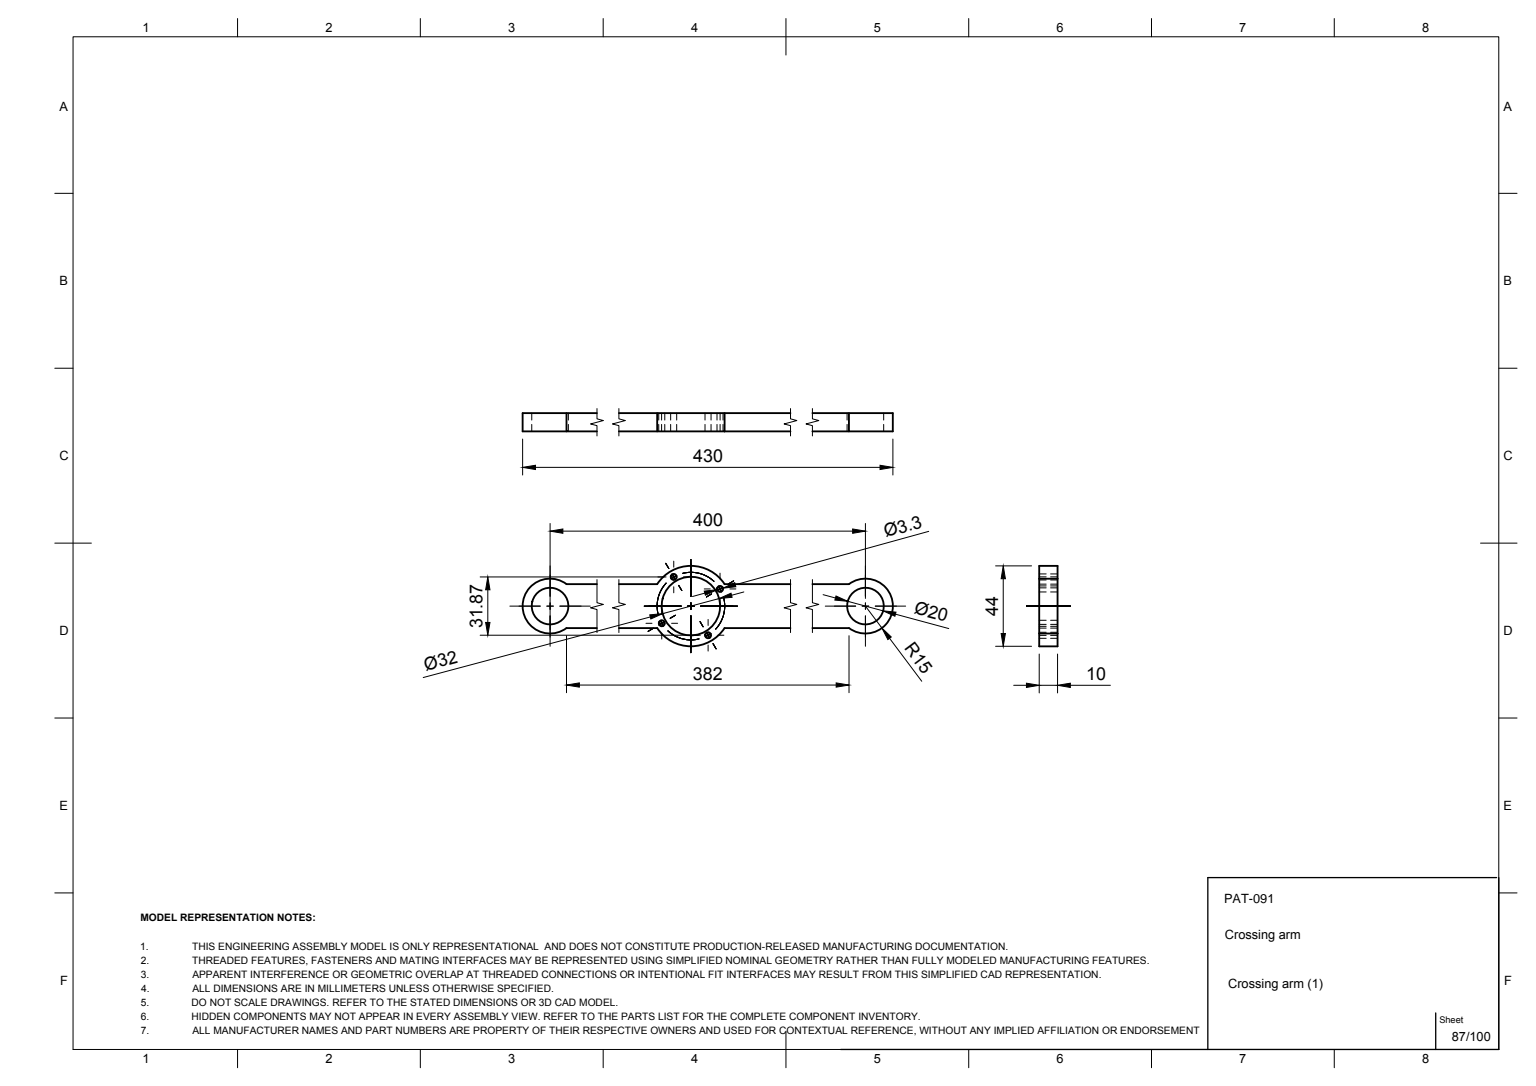
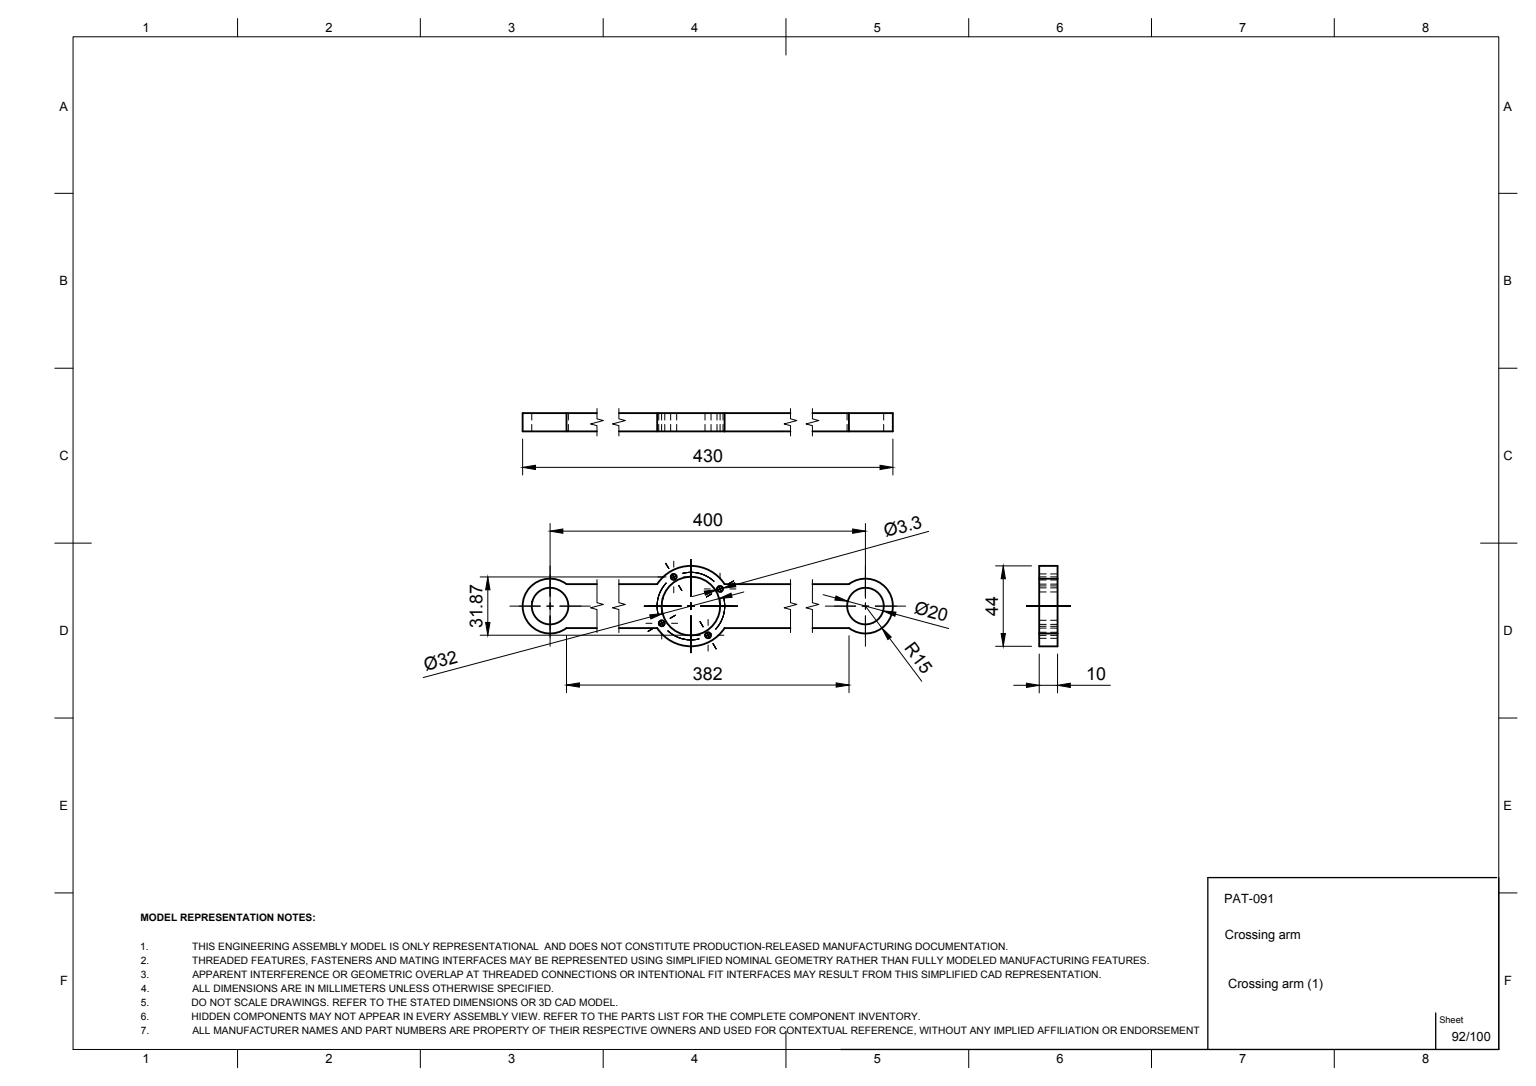
ISO-10303-21;
HEADER;
/* Generated by software containing ST-Developer
 * from STEP Tools, Inc. (www.steptools.com) 
 */

FILE_DESCRIPTION(
/* description */ ('PAT-091'),
/* implementation_level */ '2;1');

FILE_NAME(
/* name */ 'Crossing arm.step',
/* time_stamp */ '2026-10-27T15:34:44-07:00',
/* author */ (''),
/* organization */ (''),
/* preprocessor_version */ 'ST-DEVELOPER v20.2',
/* originating_system */ 'Autodesk Translation Framework v15.17.0.0',
/* authorisation */ '');

FILE_SCHEMA (('AUTOMOTIVE_DESIGN { 1 0 10303 214 3 1 1 }'));
ENDSEC;

DATA;
#10=MECHANICAL_DESIGN_GEOMETRIC_PRESENTATION_REPRESENTATION('',(#1044),#25100);
#824=SHAPE_REPRESENTATION_RELATIONSHIP('SRR','None',#25591,#934);
#934=ADVANCED_BREP_SHAPE_REPRESENTATION('',(#1165),#25061);
#1044=STYLED_ITEM('',(#26177),#1165);
#1165=MANIFOLD_SOLID_BREP('Body1',#13324);
#1525=FACE_BOUND('',#3750,.T.);
#1526=FACE_BOUND('',#3751,.T.);
#1527=FACE_BOUND('',#3752,.T.);
#1528=FACE_BOUND('',#3753,.T.);
#1529=FACE_BOUND('',#3754,.T.);
#1530=FACE_BOUND('',#3755,.T.);
#1531=FACE_BOUND('',#3756,.T.);
#1532=FACE_BOUND('',#3765,.T.);
#1533=FACE_BOUND('',#3766,.T.);
#1534=FACE_BOUND('',#3767,.T.);
#1535=FACE_BOUND('',#3768,.T.);
#1536=FACE_BOUND('',#3769,.T.);
#1537=FACE_BOUND('',#3770,.T.);
#1538=FACE_BOUND('',#3771,.T.);
#1948=PLANE('',#15794);
#1949=PLANE('',#15795);
#1950=PLANE('',#15800);
#1951=PLANE('',#15805);
#1952=PLANE('',#15810);
#1953=PLANE('',#15811);
#2613=FACE_OUTER_BOUND('',#3741,.T.);
#2614=FACE_OUTER_BOUND('',#3742,.T.);
#2615=FACE_OUTER_BOUND('',#3743,.T.);
#2616=FACE_OUTER_BOUND('',#3744,.T.);
#2617=FACE_OUTER_BOUND('',#3745,.T.);
#2618=FACE_OUTER_BOUND('',#3746,.T.);
#2619=FACE_OUTER_BOUND('',#3747,.T.);
#2620=FACE_OUTER_BOUND('',#3748,.T.);
#2621=FACE_OUTER_BOUND('',#3749,.T.);
#2622=FACE_OUTER_BOUND('',#3757,.T.);
#2623=FACE_OUTER_BOUND('',#3758,.T.);
#2624=FACE_OUTER_BOUND('',#3759,.T.);
#2625=FACE_OUTER_BOUND('',#3760,.T.);
#2626=FACE_OUTER_BOUND('',#3761,.T.);
#2627=FACE_OUTER_BOUND('',#3762,.T.);
#2628=FACE_OUTER_BOUND('',#3763,.T.);
#2629=FACE_OUTER_BOUND('',#3764,.T.);
#3741=EDGE_LOOP('',(#11144,#11145,#11146,#11147));
#3742=EDGE_LOOP('',(#11148,#11149,#11150,#11151));
#3743=EDGE_LOOP('',(#11152,#11153,#11154,#11155));
#3744=EDGE_LOOP('',(#11156,#11157,#11158,#11159));
#3745=EDGE_LOOP('',(#11160,#11161,#11162,#11163));
#3746=EDGE_LOOP('',(#11164,#11165,#11166,#11167));
#3747=EDGE_LOOP('',(#11168,#11169,#11170,#11171));
#3748=EDGE_LOOP('',(#11172,#11173,#11174,#11175));
#3749=EDGE_LOOP('',(#11176,#11177,#11178,#11179,#11180,#11181,#11182,#11183));
#3750=EDGE_LOOP('',(#11184));
#3751=EDGE_LOOP('',(#11185));
#3752=EDGE_LOOP('',(#11186));
#3753=EDGE_LOOP('',(#11187));
#3754=EDGE_LOOP('',(#11188));
#3755=EDGE_LOOP('',(#11189));
#3756=EDGE_LOOP('',(#11190));
#3757=EDGE_LOOP('',(#11191,#11192,#11193,#11194));
#3758=EDGE_LOOP('',(#11195,#11196,#11197,#11198));
#3759=EDGE_LOOP('',(#11199,#11200,#11201,#11202));
#3760=EDGE_LOOP('',(#11203,#11204,#11205,#11206));
#3761=EDGE_LOOP('',(#11207,#11208,#11209,#11210));
#3762=EDGE_LOOP('',(#11211,#11212,#11213,#11214));
#3763=EDGE_LOOP('',(#11215,#11216,#11217,#11218));
#3764=EDGE_LOOP('',(#11219,#11220,#11221,#11222,#11223,#11224,#11225,#11226));
#3765=EDGE_LOOP('',(#11227));
#3766=EDGE_LOOP('',(#11228));
#3767=EDGE_LOOP('',(#11229));
#3768=EDGE_LOOP('',(#11230));
#3769=EDGE_LOOP('',(#11231));
#3770=EDGE_LOOP('',(#11232));
#3771=EDGE_LOOP('',(#11233));
#4724=LINE('',#23542,#5464);
#4725=LINE('',#23548,#5465);
#4726=LINE('',#23554,#5466);
#4727=LINE('',#23560,#5467);
#4728=LINE('',#23566,#5468);
#4729=LINE('',#23571,#5469);
#4730=LINE('',#23575,#5470);
#4731=LINE('',#23580,#5471);
#4732=LINE('',#23584,#5472);
#4733=LINE('',#23588,#5473);
#4734=LINE('',#23590,#5474);
#4735=LINE('',#23591,#5475);
#4736=LINE('',#23595,#5476);
#4737=LINE('',#23597,#5477);
#4738=LINE('',#23600,#5478);
#4739=LINE('',#23607,#5479);
#4740=LINE('',#23608,#5480);
#4741=LINE('',#23612,#5481);
#4742=LINE('',#23615,#5482);
#4743=LINE('',#23618,#5483);
#4744=LINE('',#23620,#5484);
#4745=LINE('',#23624,#5485);
#4746=LINE('',#23628,#5486);
#5464=VECTOR('',#19448,0.164999999999999);
#5465=VECTOR('',#19455,0.164999999999999);
#5466=VECTOR('',#19462,0.164999999999999);
#5467=VECTOR('',#19469,0.164999999999999);
#5468=VECTOR('',#19476,1.6);
#5469=VECTOR('',#19481,1.);
#5470=VECTOR('',#19484,1.);
#5471=VECTOR('',#19489,1.);
#5472=VECTOR('',#19492,1.);
#5473=VECTOR('',#19497,1.);
#5474=VECTOR('',#19498,1.);
#5475=VECTOR('',#19499,1.);
#5476=VECTOR('',#19504,1.);
#5477=VECTOR('',#19505,1.);
#5478=VECTOR('',#19508,1.);
#5479=VECTOR('',#19515,1.);
#5480=VECTOR('',#19516,1.);
#5481=VECTOR('',#19521,1.);
#5482=VECTOR('',#19524,1.);
#5483=VECTOR('',#19527,1.);
#5484=VECTOR('',#19530,1.);
#5485=VECTOR('',#19535,1.);
#5486=VECTOR('',#19542,1.);
#6086=CIRCLE('',#15774,0.164999999999999);
#6087=CIRCLE('',#15775,0.164999999999999);
#6088=CIRCLE('',#15777,0.164999999999999);
#6089=CIRCLE('',#15778,0.164999999999999);
#6090=CIRCLE('',#15780,0.164999999999999);
#6091=CIRCLE('',#15781,0.164999999999999);
#6092=CIRCLE('',#15783,0.164999999999999);
#6093=CIRCLE('',#15784,0.164999999999999);
#6094=CIRCLE('',#15786,1.6);
#6095=CIRCLE('',#15787,1.6);
#6096=CIRCLE('',#15789,2.2);
#6097=CIRCLE('',#15790,2.2);
#6098=CIRCLE('',#15792,2.2);
#6099=CIRCLE('',#15793,2.2);
#6100=CIRCLE('',#15796,1.5);
#6101=CIRCLE('',#15797,1.5);
#6102=CIRCLE('',#15798,1.);
#6103=CIRCLE('',#15799,1.);
#6104=CIRCLE('',#15802,1.);
#6105=CIRCLE('',#15804,1.5);
#6106=CIRCLE('',#15807,1.);
#6107=CIRCLE('',#15809,1.5);
#7103=VERTEX_POINT('',#23539);
#7104=VERTEX_POINT('',#23541);
#7105=VERTEX_POINT('',#23545);
#7106=VERTEX_POINT('',#23547);
#7107=VERTEX_POINT('',#23551);
#7108=VERTEX_POINT('',#23553);
#7109=VERTEX_POINT('',#23557);
#7110=VERTEX_POINT('',#23559);
#7111=VERTEX_POINT('',#23563);
#7112=VERTEX_POINT('',#23565);
#7113=VERTEX_POINT('',#23569);
#7114=VERTEX_POINT('',#23570);
#7115=VERTEX_POINT('',#23572);
#7116=VERTEX_POINT('',#23574);
#7117=VERTEX_POINT('',#23578);
#7118=VERTEX_POINT('',#23579);
#7119=VERTEX_POINT('',#23581);
#7120=VERTEX_POINT('',#23583);
#7121=VERTEX_POINT('',#23587);
#7122=VERTEX_POINT('',#23589);
#7123=VERTEX_POINT('',#23593);
#7124=VERTEX_POINT('',#23596);
#7125=VERTEX_POINT('',#23598);
#7126=VERTEX_POINT('',#23601);
#7127=VERTEX_POINT('',#23603);
#7128=VERTEX_POINT('',#23606);
#7129=VERTEX_POINT('',#23610);
#7130=VERTEX_POINT('',#23614);
#7131=VERTEX_POINT('',#23616);
#7132=VERTEX_POINT('',#23622);
#8507=EDGE_CURVE('',#7103,#7103,#6086,.T.);
#8508=EDGE_CURVE('',#7103,#7104,#4724,.T.);
#8509=EDGE_CURVE('',#7104,#7104,#6087,.T.);
#8510=EDGE_CURVE('',#7105,#7105,#6088,.T.);
#8511=EDGE_CURVE('',#7105,#7106,#4725,.T.);
#8512=EDGE_CURVE('',#7106,#7106,#6089,.T.);
#8513=EDGE_CURVE('',#7107,#7107,#6090,.T.);
#8514=EDGE_CURVE('',#7107,#7108,#4726,.T.);
#8515=EDGE_CURVE('',#7108,#7108,#6091,.T.);
#8516=EDGE_CURVE('',#7109,#7109,#6092,.T.);
#8517=EDGE_CURVE('',#7109,#7110,#4727,.T.);
#8518=EDGE_CURVE('',#7110,#7110,#6093,.T.);
#8519=EDGE_CURVE('',#7111,#7111,#6094,.T.);
#8520=EDGE_CURVE('',#7111,#7112,#4728,.T.);
#8521=EDGE_CURVE('',#7112,#7112,#6095,.T.);
#8522=EDGE_CURVE('',#7113,#7114,#4729,.T.);
#8523=EDGE_CURVE('',#7115,#7113,#6096,.T.);
#8524=EDGE_CURVE('',#7116,#7115,#4730,.T.);
#8525=EDGE_CURVE('',#7116,#7114,#6097,.T.);
#8526=EDGE_CURVE('',#7117,#7118,#4731,.T.);
#8527=EDGE_CURVE('',#7117,#7119,#6098,.T.);
#8528=EDGE_CURVE('',#7120,#7119,#4732,.T.);
#8529=EDGE_CURVE('',#7118,#7120,#6099,.T.);
#8530=EDGE_CURVE('',#7119,#7121,#4733,.T.);
#8531=EDGE_CURVE('',#7121,#7122,#4734,.T.);
#8532=EDGE_CURVE('',#7120,#7122,#4735,.T.);
#8533=EDGE_CURVE('',#7122,#7123,#6100,.T.);
#8534=EDGE_CURVE('',#7123,#7115,#4736,.T.);
#8535=EDGE_CURVE('',#7113,#7124,#4737,.T.);
#8536=EDGE_CURVE('',#7124,#7125,#6101,.T.);
#8537=EDGE_CURVE('',#7125,#7118,#4738,.T.);
#8538=EDGE_CURVE('',#7126,#7126,#6102,.T.);
#8539=EDGE_CURVE('',#7127,#7127,#6103,.T.);
#8540=EDGE_CURVE('',#7123,#7128,#4739,.T.);
#8541=EDGE_CURVE('',#7128,#7116,#4740,.T.);
#8542=EDGE_CURVE('',#7129,#7129,#6104,.T.);
#8543=EDGE_CURVE('',#7129,#7126,#4741,.T.);
#8544=EDGE_CURVE('',#7130,#7124,#4742,.T.);
#8545=EDGE_CURVE('',#7130,#7131,#6105,.T.);
#8546=EDGE_CURVE('',#7125,#7131,#4743,.T.);
#8547=EDGE_CURVE('',#7114,#7130,#4744,.T.);
#8548=EDGE_CURVE('',#7132,#7132,#6106,.T.);
#8549=EDGE_CURVE('',#7132,#7127,#4745,.T.);
#8550=EDGE_CURVE('',#7121,#7128,#6107,.T.);
#8551=EDGE_CURVE('',#7131,#7117,#4746,.T.);
#11144=ORIENTED_EDGE('',*,*,#8507,.F.);
#11145=ORIENTED_EDGE('',*,*,#8508,.T.);
#11146=ORIENTED_EDGE('',*,*,#8509,.F.);
#11147=ORIENTED_EDGE('',*,*,#8508,.F.);
#11148=ORIENTED_EDGE('',*,*,#8510,.F.);
#11149=ORIENTED_EDGE('',*,*,#8511,.T.);
#11150=ORIENTED_EDGE('',*,*,#8512,.F.);
#11151=ORIENTED_EDGE('',*,*,#8511,.F.);
#11152=ORIENTED_EDGE('',*,*,#8513,.F.);
#11153=ORIENTED_EDGE('',*,*,#8514,.T.);
#11154=ORIENTED_EDGE('',*,*,#8515,.F.);
#11155=ORIENTED_EDGE('',*,*,#8514,.F.);
#11156=ORIENTED_EDGE('',*,*,#8516,.F.);
#11157=ORIENTED_EDGE('',*,*,#8517,.T.);
#11158=ORIENTED_EDGE('',*,*,#8518,.F.);
#11159=ORIENTED_EDGE('',*,*,#8517,.F.);
#11160=ORIENTED_EDGE('',*,*,#8519,.F.);
#11161=ORIENTED_EDGE('',*,*,#8520,.T.);
#11162=ORIENTED_EDGE('',*,*,#8521,.F.);
#11163=ORIENTED_EDGE('',*,*,#8520,.F.);
#11164=ORIENTED_EDGE('',*,*,#8522,.F.);
#11165=ORIENTED_EDGE('',*,*,#8523,.F.);
#11166=ORIENTED_EDGE('',*,*,#8524,.F.);
#11167=ORIENTED_EDGE('',*,*,#8525,.T.);
#11168=ORIENTED_EDGE('',*,*,#8526,.F.);
#11169=ORIENTED_EDGE('',*,*,#8527,.T.);
#11170=ORIENTED_EDGE('',*,*,#8528,.F.);
#11171=ORIENTED_EDGE('',*,*,#8529,.F.);
#11172=ORIENTED_EDGE('',*,*,#8528,.T.);
#11173=ORIENTED_EDGE('',*,*,#8530,.T.);
#11174=ORIENTED_EDGE('',*,*,#8531,.T.);
#11175=ORIENTED_EDGE('',*,*,#8532,.F.);
#11176=ORIENTED_EDGE('',*,*,#8532,.T.);
#11177=ORIENTED_EDGE('',*,*,#8533,.T.);
#11178=ORIENTED_EDGE('',*,*,#8534,.T.);
#11179=ORIENTED_EDGE('',*,*,#8523,.T.);
#11180=ORIENTED_EDGE('',*,*,#8535,.T.);
#11181=ORIENTED_EDGE('',*,*,#8536,.T.);
#11182=ORIENTED_EDGE('',*,*,#8537,.T.);
#11183=ORIENTED_EDGE('',*,*,#8529,.T.);
#11184=ORIENTED_EDGE('',*,*,#8538,.T.);
#11185=ORIENTED_EDGE('',*,*,#8539,.T.);
#11186=ORIENTED_EDGE('',*,*,#8521,.T.);
#11187=ORIENTED_EDGE('',*,*,#8518,.T.);
#11188=ORIENTED_EDGE('',*,*,#8515,.T.);
#11189=ORIENTED_EDGE('',*,*,#8512,.T.);
#11190=ORIENTED_EDGE('',*,*,#8509,.T.);
#11191=ORIENTED_EDGE('',*,*,#8524,.T.);
#11192=ORIENTED_EDGE('',*,*,#8534,.F.);
#11193=ORIENTED_EDGE('',*,*,#8540,.T.);
#11194=ORIENTED_EDGE('',*,*,#8541,.T.);
#11195=ORIENTED_EDGE('',*,*,#8542,.F.);
#11196=ORIENTED_EDGE('',*,*,#8543,.T.);
#11197=ORIENTED_EDGE('',*,*,#8538,.F.);
#11198=ORIENTED_EDGE('',*,*,#8543,.F.);
#11199=ORIENTED_EDGE('',*,*,#8544,.F.);
#11200=ORIENTED_EDGE('',*,*,#8545,.T.);
#11201=ORIENTED_EDGE('',*,*,#8546,.F.);
#11202=ORIENTED_EDGE('',*,*,#8536,.F.);
#11203=ORIENTED_EDGE('',*,*,#8522,.T.);
#11204=ORIENTED_EDGE('',*,*,#8547,.T.);
#11205=ORIENTED_EDGE('',*,*,#8544,.T.);
#11206=ORIENTED_EDGE('',*,*,#8535,.F.);
#11207=ORIENTED_EDGE('',*,*,#8548,.F.);
#11208=ORIENTED_EDGE('',*,*,#8549,.T.);
#11209=ORIENTED_EDGE('',*,*,#8539,.F.);
#11210=ORIENTED_EDGE('',*,*,#8549,.F.);
#11211=ORIENTED_EDGE('',*,*,#8531,.F.);
#11212=ORIENTED_EDGE('',*,*,#8550,.T.);
#11213=ORIENTED_EDGE('',*,*,#8540,.F.);
#11214=ORIENTED_EDGE('',*,*,#8533,.F.);
#11215=ORIENTED_EDGE('',*,*,#8526,.T.);
#11216=ORIENTED_EDGE('',*,*,#8537,.F.);
#11217=ORIENTED_EDGE('',*,*,#8546,.T.);
#11218=ORIENTED_EDGE('',*,*,#8551,.T.);
#11219=ORIENTED_EDGE('',*,*,#8551,.F.);
#11220=ORIENTED_EDGE('',*,*,#8545,.F.);
#11221=ORIENTED_EDGE('',*,*,#8547,.F.);
#11222=ORIENTED_EDGE('',*,*,#8525,.F.);
#11223=ORIENTED_EDGE('',*,*,#8541,.F.);
#11224=ORIENTED_EDGE('',*,*,#8550,.F.);
#11225=ORIENTED_EDGE('',*,*,#8530,.F.);
#11226=ORIENTED_EDGE('',*,*,#8527,.F.);
#11227=ORIENTED_EDGE('',*,*,#8542,.T.);
#11228=ORIENTED_EDGE('',*,*,#8548,.T.);
#11229=ORIENTED_EDGE('',*,*,#8519,.T.);
#11230=ORIENTED_EDGE('',*,*,#8516,.T.);
#11231=ORIENTED_EDGE('',*,*,#8513,.T.);
#11232=ORIENTED_EDGE('',*,*,#8510,.T.);
#11233=ORIENTED_EDGE('',*,*,#8507,.T.);
#12304=CYLINDRICAL_SURFACE('',#15773,0.164999999999999);
#12305=CYLINDRICAL_SURFACE('',#15776,0.164999999999999);
#12306=CYLINDRICAL_SURFACE('',#15779,0.164999999999999);
#12307=CYLINDRICAL_SURFACE('',#15782,0.164999999999999);
#12308=CYLINDRICAL_SURFACE('',#15785,1.6);
#12309=CYLINDRICAL_SURFACE('',#15788,2.2);
#12310=CYLINDRICAL_SURFACE('',#15791,2.2);
#12311=CYLINDRICAL_SURFACE('',#15801,1.);
#12312=CYLINDRICAL_SURFACE('',#15803,1.5);
#12313=CYLINDRICAL_SURFACE('',#15806,1.);
#12314=CYLINDRICAL_SURFACE('',#15808,1.5);
#12980=ADVANCED_FACE('',(#2613),#12304,.F.);
#12981=ADVANCED_FACE('',(#2614),#12305,.F.);
#12982=ADVANCED_FACE('',(#2615),#12306,.F.);
#12983=ADVANCED_FACE('',(#2616),#12307,.F.);
#12984=ADVANCED_FACE('',(#2617),#12308,.F.);
#12985=ADVANCED_FACE('',(#2618),#12309,.T.);
#12986=ADVANCED_FACE('',(#2619),#12310,.T.);
#12987=ADVANCED_FACE('',(#2620),#1948,.T.);
#12988=ADVANCED_FACE('',(#2621,#1525,#1526,#1527,#1528,#1529,#1530,#1531),
#1949,.T.);
#12989=ADVANCED_FACE('',(#2622),#1950,.T.);
#12990=ADVANCED_FACE('',(#2623),#12311,.F.);
#12991=ADVANCED_FACE('',(#2624),#12312,.T.);
#12992=ADVANCED_FACE('',(#2625),#1951,.T.);
#12993=ADVANCED_FACE('',(#2626),#12313,.F.);
#12994=ADVANCED_FACE('',(#2627),#12314,.T.);
#12995=ADVANCED_FACE('',(#2628),#1952,.T.);
#12996=ADVANCED_FACE('',(#2629,#1532,#1533,#1534,#1535,#1536,#1537,#1538),
#1953,.F.);
#13324=CLOSED_SHELL('',(#12980,#12981,#12982,#12983,#12984,#12985,#12986,
#12987,#12988,#12989,#12990,#12991,#12992,#12993,#12994,#12995,#12996));
#15772=AXIS2_PLACEMENT_3D('',#23537,#19442,#19443);
#15773=AXIS2_PLACEMENT_3D('',#23538,#19444,#19445);
#15774=AXIS2_PLACEMENT_3D('',#23540,#19446,#19447);
#15775=AXIS2_PLACEMENT_3D('',#23543,#19449,#19450);
#15776=AXIS2_PLACEMENT_3D('',#23544,#19451,#19452);
#15777=AXIS2_PLACEMENT_3D('',#23546,#19453,#19454);
#15778=AXIS2_PLACEMENT_3D('',#23549,#19456,#19457);
#15779=AXIS2_PLACEMENT_3D('',#23550,#19458,#19459);
#15780=AXIS2_PLACEMENT_3D('',#23552,#19460,#19461);
#15781=AXIS2_PLACEMENT_3D('',#23555,#19463,#19464);
#15782=AXIS2_PLACEMENT_3D('',#23556,#19465,#19466);
#15783=AXIS2_PLACEMENT_3D('',#23558,#19467,#19468);
#15784=AXIS2_PLACEMENT_3D('',#23561,#19470,#19471);
#15785=AXIS2_PLACEMENT_3D('',#23562,#19472,#19473);
#15786=AXIS2_PLACEMENT_3D('',#23564,#19474,#19475);
#15787=AXIS2_PLACEMENT_3D('',#23567,#19477,#19478);
#15788=AXIS2_PLACEMENT_3D('',#23568,#19479,#19480);
#15789=AXIS2_PLACEMENT_3D('',#23573,#19482,#19483);
#15790=AXIS2_PLACEMENT_3D('',#23576,#19485,#19486);
#15791=AXIS2_PLACEMENT_3D('',#23577,#19487,#19488);
#15792=AXIS2_PLACEMENT_3D('',#23582,#19490,#19491);
#15793=AXIS2_PLACEMENT_3D('',#23585,#19493,#19494);
#15794=AXIS2_PLACEMENT_3D('',#23586,#19495,#19496);
#15795=AXIS2_PLACEMENT_3D('',#23592,#19500,#19501);
#15796=AXIS2_PLACEMENT_3D('',#23594,#19502,#19503);
#15797=AXIS2_PLACEMENT_3D('',#23599,#19506,#19507);
#15798=AXIS2_PLACEMENT_3D('',#23602,#19509,#19510);
#15799=AXIS2_PLACEMENT_3D('',#23604,#19511,#19512);
#15800=AXIS2_PLACEMENT_3D('',#23605,#19513,#19514);
#15801=AXIS2_PLACEMENT_3D('',#23609,#19517,#19518);
#15802=AXIS2_PLACEMENT_3D('',#23611,#19519,#19520);
#15803=AXIS2_PLACEMENT_3D('',#23613,#19522,#19523);
#15804=AXIS2_PLACEMENT_3D('',#23617,#19525,#19526);
#15805=AXIS2_PLACEMENT_3D('',#23619,#19528,#19529);
#15806=AXIS2_PLACEMENT_3D('',#23621,#19531,#19532);
#15807=AXIS2_PLACEMENT_3D('',#23623,#19533,#19534);
#15808=AXIS2_PLACEMENT_3D('',#23625,#19536,#19537);
#15809=AXIS2_PLACEMENT_3D('',#23626,#19538,#19539);
#15810=AXIS2_PLACEMENT_3D('',#23627,#19540,#19541);
#15811=AXIS2_PLACEMENT_3D('',#23629,#19543,#19544);
#19442=DIRECTION('axis',(0.,0.,1.));
#19443=DIRECTION('refdir',(1.,0.,0.));
#19444=DIRECTION('center_axis',(0.,1.,0.));
#19445=DIRECTION('ref_axis',(1.,0.,0.));
#19446=DIRECTION('center_axis',(0.,1.,0.));
#19447=DIRECTION('ref_axis',(1.,0.,0.));
#19448=DIRECTION('',(0.,1.,0.));
#19449=DIRECTION('center_axis',(0.,-1.,0.));
#19450=DIRECTION('ref_axis',(1.,0.,0.));
#19451=DIRECTION('center_axis',(0.,1.,0.));
#19452=DIRECTION('ref_axis',(1.,0.,0.));
#19453=DIRECTION('center_axis',(0.,1.,0.));
#19454=DIRECTION('ref_axis',(1.,0.,0.));
#19455=DIRECTION('',(0.,1.,0.));
#19456=DIRECTION('center_axis',(0.,-1.,0.));
#19457=DIRECTION('ref_axis',(1.,0.,0.));
#19458=DIRECTION('center_axis',(0.,1.,0.));
#19459=DIRECTION('ref_axis',(1.,0.,0.));
#19460=DIRECTION('center_axis',(0.,1.,0.));
#19461=DIRECTION('ref_axis',(1.,0.,0.));
#19462=DIRECTION('',(0.,1.,0.));
#19463=DIRECTION('center_axis',(0.,-1.,0.));
#19464=DIRECTION('ref_axis',(1.,0.,0.));
#19465=DIRECTION('center_axis',(0.,1.,0.));
#19466=DIRECTION('ref_axis',(1.,0.,0.));
#19467=DIRECTION('center_axis',(0.,1.,0.));
#19468=DIRECTION('ref_axis',(1.,0.,0.));
#19469=DIRECTION('',(0.,1.,0.));
#19470=DIRECTION('center_axis',(0.,-1.,0.));
#19471=DIRECTION('ref_axis',(1.,0.,0.));
#19472=DIRECTION('center_axis',(0.,1.,0.));
#19473=DIRECTION('ref_axis',(1.,0.,0.));
#19474=DIRECTION('center_axis',(0.,1.,0.));
#19475=DIRECTION('ref_axis',(1.,0.,0.));
#19476=DIRECTION('',(0.,1.,0.));
#19477=DIRECTION('center_axis',(0.,-1.,0.));
#19478=DIRECTION('ref_axis',(1.,0.,0.));
#19479=DIRECTION('center_axis',(0.,1.,0.));
#19480=DIRECTION('ref_axis',(1.,0.,0.));
#19481=DIRECTION('',(0.,-1.,0.));
#19482=DIRECTION('center_axis',(0.,1.,0.));
#19483=DIRECTION('ref_axis',(1.,0.,0.));
#19484=DIRECTION('',(0.,1.,0.));
#19485=DIRECTION('center_axis',(0.,1.,0.));
#19486=DIRECTION('ref_axis',(1.,0.,0.));
#19487=DIRECTION('center_axis',(0.,1.,0.));
#19488=DIRECTION('ref_axis',(1.,0.,0.));
#19489=DIRECTION('',(0.,1.,0.));
#19490=DIRECTION('center_axis',(0.,1.,0.));
#19491=DIRECTION('ref_axis',(1.,0.,0.));
#19492=DIRECTION('',(0.,-1.,0.));
#19493=DIRECTION('center_axis',(0.,1.,0.));
#19494=DIRECTION('ref_axis',(1.,0.,0.));
#19495=DIRECTION('center_axis',(0.25,0.,0.968245836551854));
#19496=DIRECTION('ref_axis',(0.968245836551854,0.,-0.25));
#19497=DIRECTION('',(0.968245836551854,0.,-0.25));
#19498=DIRECTION('',(0.,1.,0.));
#19499=DIRECTION('',(0.968245836551854,0.,-0.25));
#19500=DIRECTION('center_axis',(0.,1.,0.));
#19501=DIRECTION('ref_axis',(0.,0.,1.));
#19502=DIRECTION('center_axis',(0.,1.,0.));
#19503=DIRECTION('ref_axis',(1.,0.,0.));
#19504=DIRECTION('',(-0.968245836551854,0.,0.25));
#19505=DIRECTION('',(-0.968245836551854,0.,0.25));
#19506=DIRECTION('center_axis',(0.,1.,0.));
#19507=DIRECTION('ref_axis',(1.,0.,0.));
#19508=DIRECTION('',(0.968245836551854,0.,-0.25));
#19509=DIRECTION('center_axis',(0.,-1.,0.));
#19510=DIRECTION('ref_axis',(1.,0.,0.));
#19511=DIRECTION('center_axis',(0.,-1.,0.));
#19512=DIRECTION('ref_axis',(1.,0.,0.));
#19513=DIRECTION('center_axis',(-0.25,0.,-0.968245836551854));
#19514=DIRECTION('ref_axis',(-0.968245836551854,0.,0.25));
#19515=DIRECTION('',(0.,-1.,0.));
#19516=DIRECTION('',(-0.968245836551854,0.,0.25));
#19517=DIRECTION('center_axis',(0.,1.,0.));
#19518=DIRECTION('ref_axis',(1.,0.,0.));
#19519=DIRECTION('center_axis',(0.,1.,0.));
#19520=DIRECTION('ref_axis',(1.,0.,0.));
#19521=DIRECTION('',(0.,1.,0.));
#19522=DIRECTION('center_axis',(0.,1.,0.));
#19523=DIRECTION('ref_axis',(-0.968245836551855,0.,0.249999999999998));
#19524=DIRECTION('',(0.,1.,0.));
#19525=DIRECTION('center_axis',(0.,1.,0.));
#19526=DIRECTION('ref_axis',(1.,0.,0.));
#19527=DIRECTION('',(0.,-1.,0.));
#19528=DIRECTION('center_axis',(-0.25,0.,-0.968245836551854));
#19529=DIRECTION('ref_axis',(-0.968245836551854,0.,0.25));
#19530=DIRECTION('',(-0.968245836551854,0.,0.25));
#19531=DIRECTION('center_axis',(0.,1.,0.));
#19532=DIRECTION('ref_axis',(1.,0.,0.));
#19533=DIRECTION('center_axis',(0.,1.,0.));
#19534=DIRECTION('ref_axis',(1.,0.,0.));
#19535=DIRECTION('',(0.,1.,0.));
#19536=DIRECTION('center_axis',(0.,1.,0.));
#19537=DIRECTION('ref_axis',(1.,0.,0.));
#19538=DIRECTION('center_axis',(0.,1.,0.));
#19539=DIRECTION('ref_axis',(1.,0.,0.));
#19540=DIRECTION('center_axis',(0.25,0.,0.968245836551854));
#19541=DIRECTION('ref_axis',(0.968245836551854,0.,-0.25));
#19542=DIRECTION('',(0.968245836551854,0.,-0.25));
#19543=DIRECTION('center_axis',(0.,1.,0.));
#19544=DIRECTION('ref_axis',(1.,0.,0.));
#23537=CARTESIAN_POINT('',(0.,0.,0.));
#23538=CARTESIAN_POINT('Origin',(18.056769185842,-5.6,6.69185245480489));
#23539=CARTESIAN_POINT('',(17.891769185842,-5.5,6.69185245480489));
#23540=CARTESIAN_POINT('Origin',(18.056769185842,-5.5,6.69185245480489));
#23541=CARTESIAN_POINT('',(17.891769185842,-4.5,6.69185245480489));
#23542=CARTESIAN_POINT('',(17.891769185842,-5.6,6.69185245480489));
#23543=CARTESIAN_POINT('Origin',(18.056769185842,-4.5,6.69185245480489));
#23544=CARTESIAN_POINT('Origin',(18.056769185842,-5.6,9.30814754519511));
#23545=CARTESIAN_POINT('',(17.891769185842,-5.5,9.30814754519511));
#23546=CARTESIAN_POINT('Origin',(18.056769185842,-5.5,9.30814754519511));
#23547=CARTESIAN_POINT('',(17.891769185842,-4.5,9.30814754519511));
#23548=CARTESIAN_POINT('',(17.891769185842,-5.6,9.30814754519511));
#23549=CARTESIAN_POINT('Origin',(18.056769185842,-4.5,9.30814754519511));
#23550=CARTESIAN_POINT('Origin',(20.6730642762322,-5.6,9.30814754519511));
#23551=CARTESIAN_POINT('',(20.5080642762322,-5.5,9.30814754519511));
#23552=CARTESIAN_POINT('Origin',(20.6730642762322,-5.5,9.30814754519511));
#23553=CARTESIAN_POINT('',(20.5080642762322,-4.5,9.30814754519511));
#23554=CARTESIAN_POINT('',(20.5080642762322,-5.6,9.30814754519511));
#23555=CARTESIAN_POINT('Origin',(20.6730642762322,-4.5,9.30814754519511));
#23556=CARTESIAN_POINT('Origin',(20.6730642762322,-5.6,6.69185245480489));
#23557=CARTESIAN_POINT('',(20.5080642762322,-5.5,6.69185245480489));
#23558=CARTESIAN_POINT('Origin',(20.6730642762322,-5.5,6.69185245480489));
#23559=CARTESIAN_POINT('',(20.5080642762322,-4.5,6.69185245480489));
#23560=CARTESIAN_POINT('',(20.5080642762322,-5.6,6.69185245480489));
#23561=CARTESIAN_POINT('Origin',(20.6730642762322,-4.5,6.69185245480489));
#23562=CARTESIAN_POINT('Origin',(19.3649167310371,-5.6,8.));
#23563=CARTESIAN_POINT('',(17.7649167310371,-5.5,8.));
#23564=CARTESIAN_POINT('Origin',(19.3649167310371,-5.5,8.));
#23565=CARTESIAN_POINT('',(17.7649167310371,-4.5,8.));
#23566=CARTESIAN_POINT('',(17.7649167310371,-5.6,8.));
#23567=CARTESIAN_POINT('Origin',(19.3649167310371,-4.5,8.));
#23568=CARTESIAN_POINT('Origin',(19.3649167310371,-5.5,8.));
#23569=CARTESIAN_POINT('',(17.2795596239014,-4.5,7.29908221900242));
#23570=CARTESIAN_POINT('',(17.2795596239014,-5.5,7.29908221900242));
#23571=CARTESIAN_POINT('',(17.2795596239014,-5.5,7.29908221900242));
#23572=CARTESIAN_POINT('',(20.8502738381728,-4.5,6.37712777327313));
#23573=CARTESIAN_POINT('Origin',(19.3649167310371,-4.5,8.));
#23574=CARTESIAN_POINT('',(20.8502738381728,-5.5,6.37712777327313));
#23575=CARTESIAN_POINT('',(20.8502738381728,-5.5,6.37712777327313));
#23576=CARTESIAN_POINT('Origin',(19.3649167310371,-5.5,8.));
#23577=CARTESIAN_POINT('Origin',(19.3649167310371,-5.5,8.));
#23578=CARTESIAN_POINT('',(17.8795596239014,-5.5,9.62287222672687));
#23579=CARTESIAN_POINT('',(17.8795596239014,-4.5,9.62287222672687));
#23580=CARTESIAN_POINT('',(17.8795596239014,-5.5,9.62287222672687));
#23581=CARTESIAN_POINT('',(21.4502738381728,-5.5,8.70091778099758));
#23582=CARTESIAN_POINT('Origin',(19.3649167310371,-5.5,8.));
#23583=CARTESIAN_POINT('',(21.4502738381728,-4.5,8.70091778099758));
#23584=CARTESIAN_POINT('',(21.4502738381728,-5.5,8.70091778099758));
#23585=CARTESIAN_POINT('Origin',(19.3649167310371,-4.5,8.));
#23586=CARTESIAN_POINT('Origin',(0.3,-5.5,14.1618950038622));
#23587=CARTESIAN_POINT('',(38.1584122091775,-5.5,4.38689500386223));
#23588=CARTESIAN_POINT('',(0.3,-5.5,14.1618950038622));
#23589=CARTESIAN_POINT('',(38.1584122091775,-4.5,4.38689500386223));
#23590=CARTESIAN_POINT('',(38.1584122091775,-5.5,4.38689500386223));
#23591=CARTESIAN_POINT('',(0.3,-4.5,14.1618950038622));
#23592=CARTESIAN_POINT('Origin',(19.3649167310371,-4.5,8.));
#23593=CARTESIAN_POINT('',(37.5584122091775,-4.5,2.06310499613778));
#23594=CARTESIAN_POINT('Origin',(38.7298334620742,-4.5,3.));
#23595=CARTESIAN_POINT('',(38.4298334620742,-4.5,1.83810499613777));
#23596=CARTESIAN_POINT('',(0.571421252896674,-4.5,11.6131049961378));
#23597=CARTESIAN_POINT('',(38.4298334620742,-4.5,1.83810499613777));
#23598=CARTESIAN_POINT('',(1.17142125289667,-4.5,13.9368950038622));
#23599=CARTESIAN_POINT('Origin',(0.,-4.5,13.));
#23600=CARTESIAN_POINT('',(0.3,-4.5,14.1618950038622));
#23601=CARTESIAN_POINT('',(-1.,-4.5,13.));
#23602=CARTESIAN_POINT('Origin',(0.,-4.5,13.));
#23603=CARTESIAN_POINT('',(37.7298334620742,-4.5,3.));
#23604=CARTESIAN_POINT('Origin',(38.7298334620742,-4.5,3.));
#23605=CARTESIAN_POINT('Origin',(38.4298334620742,-5.5,1.83810499613777));
#23606=CARTESIAN_POINT('',(37.5584122091775,-5.5,2.06310499613778));
#23607=CARTESIAN_POINT('',(37.5584122091775,-5.5,2.06310499613778));
#23608=CARTESIAN_POINT('',(38.4298334620742,-5.5,1.83810499613777));
#23609=CARTESIAN_POINT('Origin',(0.,-5.6,13.));
#23610=CARTESIAN_POINT('',(-1.,-5.5,13.));
#23611=CARTESIAN_POINT('Origin',(0.,-5.5,13.));
#23612=CARTESIAN_POINT('',(-1.,-5.6,13.));
#23613=CARTESIAN_POINT('Origin',(0.,-5.5,13.));
#23614=CARTESIAN_POINT('',(0.571421252896672,-5.5,11.6131049961378));
#23615=CARTESIAN_POINT('',(0.571421252896672,-5.5,11.6131049961378));
#23616=CARTESIAN_POINT('',(1.17142125289667,-5.5,13.9368950038622));
#23617=CARTESIAN_POINT('Origin',(0.,-5.5,13.));
#23618=CARTESIAN_POINT('',(1.17142125289667,-5.5,13.9368950038622));
#23619=CARTESIAN_POINT('Origin',(38.4298334620742,-5.5,1.83810499613777));
#23620=CARTESIAN_POINT('',(38.4298334620742,-5.5,1.83810499613777));
#23621=CARTESIAN_POINT('Origin',(38.7298334620742,-5.6,3.));
#23622=CARTESIAN_POINT('',(37.7298334620742,-5.5,3.));
#23623=CARTESIAN_POINT('Origin',(38.7298334620742,-5.5,3.));
#23624=CARTESIAN_POINT('',(37.7298334620742,-5.6,3.));
#23625=CARTESIAN_POINT('Origin',(38.7298334620742,-5.5,3.));
#23626=CARTESIAN_POINT('Origin',(38.7298334620742,-5.5,3.));
#23627=CARTESIAN_POINT('Origin',(0.3,-5.5,14.1618950038622));
#23628=CARTESIAN_POINT('',(0.3,-5.5,14.1618950038622));
#23629=CARTESIAN_POINT('Origin',(19.3649167310371,-5.5,8.));
#24940=UNCERTAINTY_MEASURE_WITH_UNIT(LENGTH_MEASURE(0.001),#25101,
'DISTANCE_ACCURACY_VALUE',
'Maximum model space distance between geometric entities at asserted c
onnectivities');
#24979=UNCERTAINTY_MEASURE_WITH_UNIT(LENGTH_MEASURE(0.001),#25101,
'DISTANCE_ACCURACY_VALUE',
'Maximum model space distance between geometric entities at asserted c
onnectivities');
#25061=(
GEOMETRIC_REPRESENTATION_CONTEXT(3)
GLOBAL_UNCERTAINTY_ASSIGNED_CONTEXT((#24940))
GLOBAL_UNIT_ASSIGNED_CONTEXT((#25101,#25103,#25104))
REPRESENTATION_CONTEXT('','3D')
);
#25100=(
GEOMETRIC_REPRESENTATION_CONTEXT(3)
GLOBAL_UNCERTAINTY_ASSIGNED_CONTEXT((#24979))
GLOBAL_UNIT_ASSIGNED_CONTEXT((#25101,#25103,#25104))
REPRESENTATION_CONTEXT('','3D')
);
#25101=(
LENGTH_UNIT()
NAMED_UNIT(*)
SI_UNIT(.CENTI.,.METRE.)
);
#25103=(
NAMED_UNIT(*)
PLANE_ANGLE_UNIT()
SI_UNIT($,.RADIAN.)
);
#25104=(
NAMED_UNIT(*)
SI_UNIT($,.STERADIAN.)
SOLID_ANGLE_UNIT()
);
#25186=SHAPE_DEFINITION_REPRESENTATION(#25380,#25591);
#25380=PRODUCT_DEFINITION_SHAPE('',$,#25712);
#25591=SHAPE_REPRESENTATION('',(#15772),#25061);
#25630=PRODUCT_DEFINITION_CONTEXT('part definition',#25992,'design');
#25712=PRODUCT_DEFINITION('Crossing arm','Crossing arm',#25832,#25630);
#25832=PRODUCT_DEFINITION_FORMATION('',$,#26075);
#25992=APPLICATION_CONTEXT(
'Core Data for Automotive Mechanical Design Process');
#25993=PRODUCT_CONTEXT('part definition',#25992,'mechanical');
#26075=PRODUCT('Crossing arm','Crossing arm','Crossing arm',(#25993));
#26171=COLOUR_RGB('Light Blue',0.38,0.62,0.78);
#26172=FILL_AREA_STYLE_COLOUR('',#26171);
#26173=FILL_AREA_STYLE('',(#26172));
#26174=SURFACE_STYLE_FILL_AREA(#26173);
#26175=SURFACE_SIDE_STYLE('',(#26174));
#26176=SURFACE_STYLE_USAGE(.BOTH.,#26175);
#26177=PRESENTATION_STYLE_ASSIGNMENT((#26176));
ENDSEC;
END-ISO-10303-21;
